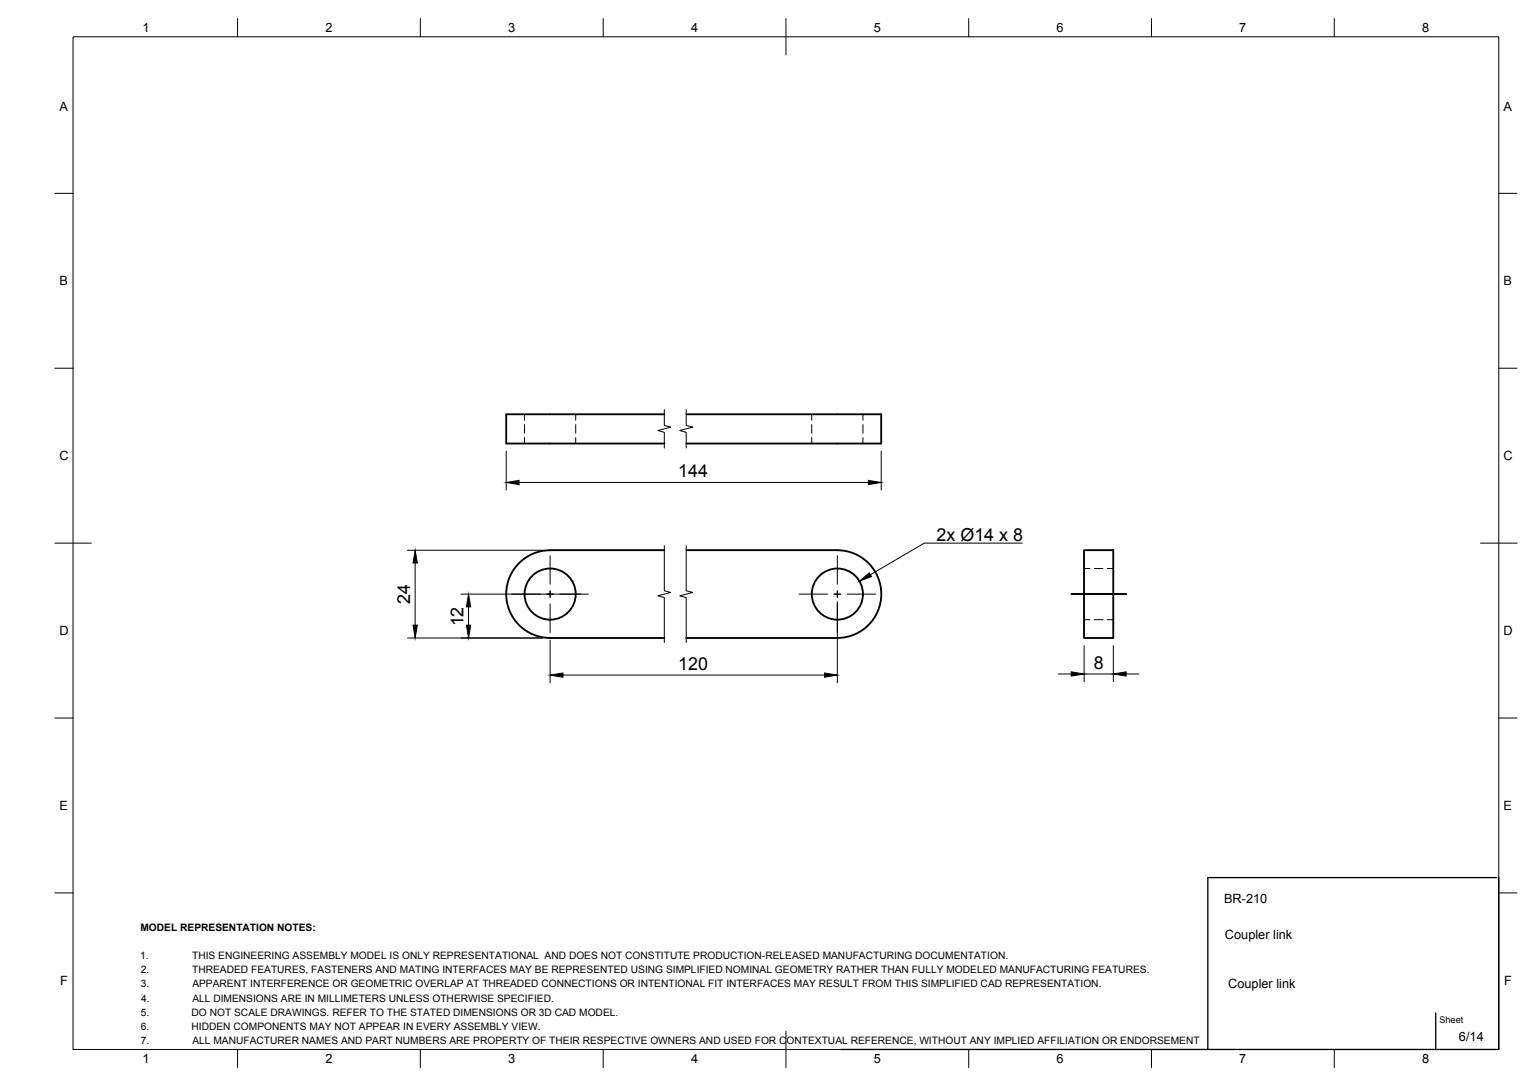
ISO-10303-21;
HEADER;
/* Generated by software containing ST-Developer
 * from STEP Tools, Inc. (www.steptools.com) 
 */

FILE_DESCRIPTION(
/* description */ ('Independent 1:2 reduction pantograph. 120 mm parallelogram sides; fix
ed fulcrum on the extension of a 240 mm link. Drawing point halfway al
ong its link, so its XY displacement is one half of the tracing point.
 Replaceable pivot bushes and retained pins. Calibration and productio
n accuracy unassigned.'),
/* implementation_level */ '2;1');

FILE_NAME(
/* name */ 'Coupler link.step',
/* time_stamp */ '2026-11-07T22:11:57-08:00',
/* author */ (''),
/* organization */ (''),
/* preprocessor_version */ 'ST-DEVELOPER v20.2',
/* originating_system */ 'Autodesk Translation Framework v15.17.0.0',
/* authorisation */ '');

FILE_SCHEMA (('AUTOMOTIVE_DESIGN { 1 0 10303 214 3 1 1 }'));
ENDSEC;

DATA;
#10=MECHANICAL_DESIGN_GEOMETRIC_PRESENTATION_REPRESENTATION('',(#193),#2926);
#167=SHAPE_REPRESENTATION_RELATIONSHIP('SRR','None',#3004,#180);
#180=ADVANCED_BREP_SHAPE_REPRESENTATION('',(#206),#2920);
#193=STYLED_ITEM('',(#3077),#206);
#206=MANIFOLD_SOLID_BREP('Body1',#1548);
#247=FACE_BOUND('',#497,.T.);
#248=FACE_BOUND('',#498,.T.);
#249=FACE_BOUND('',#500,.T.);
#250=FACE_BOUND('',#501,.T.);
#287=PLANE('',#1829);
#288=PLANE('',#1833);
#289=PLANE('',#1837);
#290=PLANE('',#1838);
#363=FACE_OUTER_BOUND('',#490,.T.);
#364=FACE_OUTER_BOUND('',#491,.T.);
#365=FACE_OUTER_BOUND('',#492,.T.);
#366=FACE_OUTER_BOUND('',#493,.T.);
#367=FACE_OUTER_BOUND('',#494,.T.);
#368=FACE_OUTER_BOUND('',#495,.T.);
#369=FACE_OUTER_BOUND('',#496,.T.);
#370=FACE_OUTER_BOUND('',#499,.T.);
#490=EDGE_LOOP('',(#1289,#1290,#1291,#1292));
#491=EDGE_LOOP('',(#1293,#1294,#1295,#1296));
#492=EDGE_LOOP('',(#1297,#1298,#1299,#1300));
#493=EDGE_LOOP('',(#1301,#1302,#1303,#1304));
#494=EDGE_LOOP('',(#1305,#1306,#1307,#1308));
#495=EDGE_LOOP('',(#1309,#1310,#1311,#1312));
#496=EDGE_LOOP('',(#1313,#1314,#1315,#1316));
#497=EDGE_LOOP('',(#1317));
#498=EDGE_LOOP('',(#1318));
#499=EDGE_LOOP('',(#1319,#1320,#1321,#1322));
#500=EDGE_LOOP('',(#1323));
#501=EDGE_LOOP('',(#1324));
#588=LINE('',#2728,#669);
#589=LINE('',#2734,#670);
#590=LINE('',#2739,#671);
#591=LINE('',#2741,#672);
#592=LINE('',#2743,#673);
#593=LINE('',#2744,#674);
#594=LINE('',#2750,#675);
#595=LINE('',#2753,#676);
#596=LINE('',#2755,#677);
#597=LINE('',#2756,#678);
#669=VECTOR('',#2236,7.);
#670=VECTOR('',#2243,7.);
#671=VECTOR('',#2248,10.);
#672=VECTOR('',#2249,10.);
#673=VECTOR('',#2250,10.);
#674=VECTOR('',#2251,10.);
#675=VECTOR('',#2258,10.);
#676=VECTOR('',#2261,10.);
#677=VECTOR('',#2262,10.);
#678=VECTOR('',#2263,10.);
#755=CIRCLE('',#1824,7.);
#756=CIRCLE('',#1825,7.);
#757=CIRCLE('',#1827,7.);
#758=CIRCLE('',#1828,7.);
#759=CIRCLE('',#1831,12.);
#760=CIRCLE('',#1832,12.);
#761=CIRCLE('',#1835,12.);
#762=CIRCLE('',#1836,12.);
#859=VERTEX_POINT('',#2725);
#860=VERTEX_POINT('',#2727);
#861=VERTEX_POINT('',#2731);
#862=VERTEX_POINT('',#2733);
#863=VERTEX_POINT('',#2737);
#864=VERTEX_POINT('',#2738);
#865=VERTEX_POINT('',#2740);
#866=VERTEX_POINT('',#2742);
#867=VERTEX_POINT('',#2746);
#868=VERTEX_POINT('',#2748);
#869=VERTEX_POINT('',#2752);
#870=VERTEX_POINT('',#2754);
#1009=EDGE_CURVE('',#859,#859,#755,.T.);
#1010=EDGE_CURVE('',#859,#860,#588,.T.);
#1011=EDGE_CURVE('',#860,#860,#756,.T.);
#1012=EDGE_CURVE('',#861,#861,#757,.T.);
#1013=EDGE_CURVE('',#861,#862,#589,.T.);
#1014=EDGE_CURVE('',#862,#862,#758,.T.);
#1015=EDGE_CURVE('',#863,#864,#590,.T.);
#1016=EDGE_CURVE('',#864,#865,#591,.T.);
#1017=EDGE_CURVE('',#866,#865,#592,.T.);
#1018=EDGE_CURVE('',#863,#866,#593,.T.);
#1019=EDGE_CURVE('',#867,#863,#759,.T.);
#1020=EDGE_CURVE('',#868,#866,#760,.T.);
#1021=EDGE_CURVE('',#867,#868,#594,.T.);
#1022=EDGE_CURVE('',#869,#867,#595,.T.);
#1023=EDGE_CURVE('',#870,#868,#596,.T.);
#1024=EDGE_CURVE('',#869,#870,#597,.T.);
#1025=EDGE_CURVE('',#864,#869,#761,.T.);
#1026=EDGE_CURVE('',#865,#870,#762,.T.);
#1289=ORIENTED_EDGE('',*,*,#1009,.F.);
#1290=ORIENTED_EDGE('',*,*,#1010,.T.);
#1291=ORIENTED_EDGE('',*,*,#1011,.F.);
#1292=ORIENTED_EDGE('',*,*,#1010,.F.);
#1293=ORIENTED_EDGE('',*,*,#1012,.F.);
#1294=ORIENTED_EDGE('',*,*,#1013,.T.);
#1295=ORIENTED_EDGE('',*,*,#1014,.F.);
#1296=ORIENTED_EDGE('',*,*,#1013,.F.);
#1297=ORIENTED_EDGE('',*,*,#1015,.T.);
#1298=ORIENTED_EDGE('',*,*,#1016,.T.);
#1299=ORIENTED_EDGE('',*,*,#1017,.F.);
#1300=ORIENTED_EDGE('',*,*,#1018,.F.);
#1301=ORIENTED_EDGE('',*,*,#1019,.T.);
#1302=ORIENTED_EDGE('',*,*,#1018,.T.);
#1303=ORIENTED_EDGE('',*,*,#1020,.F.);
#1304=ORIENTED_EDGE('',*,*,#1021,.F.);
#1305=ORIENTED_EDGE('',*,*,#1022,.T.);
#1306=ORIENTED_EDGE('',*,*,#1021,.T.);
#1307=ORIENTED_EDGE('',*,*,#1023,.F.);
#1308=ORIENTED_EDGE('',*,*,#1024,.F.);
#1309=ORIENTED_EDGE('',*,*,#1025,.T.);
#1310=ORIENTED_EDGE('',*,*,#1024,.T.);
#1311=ORIENTED_EDGE('',*,*,#1026,.F.);
#1312=ORIENTED_EDGE('',*,*,#1016,.F.);
#1313=ORIENTED_EDGE('',*,*,#1026,.T.);
#1314=ORIENTED_EDGE('',*,*,#1023,.T.);
#1315=ORIENTED_EDGE('',*,*,#1020,.T.);
#1316=ORIENTED_EDGE('',*,*,#1017,.T.);
#1317=ORIENTED_EDGE('',*,*,#1009,.T.);
#1318=ORIENTED_EDGE('',*,*,#1012,.T.);
#1319=ORIENTED_EDGE('',*,*,#1025,.F.);
#1320=ORIENTED_EDGE('',*,*,#1015,.F.);
#1321=ORIENTED_EDGE('',*,*,#1019,.F.);
#1322=ORIENTED_EDGE('',*,*,#1022,.F.);
#1323=ORIENTED_EDGE('',*,*,#1011,.T.);
#1324=ORIENTED_EDGE('',*,*,#1014,.T.);
#1434=CYLINDRICAL_SURFACE('',#1823,7.);
#1435=CYLINDRICAL_SURFACE('',#1826,7.);
#1436=CYLINDRICAL_SURFACE('',#1830,12.);
#1437=CYLINDRICAL_SURFACE('',#1834,12.);
#1507=ADVANCED_FACE('',(#363),#1434,.F.);
#1508=ADVANCED_FACE('',(#364),#1435,.F.);
#1509=ADVANCED_FACE('',(#365),#287,.T.);
#1510=ADVANCED_FACE('',(#366),#1436,.T.);
#1511=ADVANCED_FACE('',(#367),#288,.T.);
#1512=ADVANCED_FACE('',(#368),#1437,.T.);
#1513=ADVANCED_FACE('',(#369,#247,#248),#289,.T.);
#1514=ADVANCED_FACE('',(#370,#249,#250),#290,.F.);
#1548=CLOSED_SHELL('',(#1507,#1508,#1509,#1510,#1511,#1512,#1513,#1514));
#1822=AXIS2_PLACEMENT_3D('',#2723,#2230,#2231);
#1823=AXIS2_PLACEMENT_3D('',#2724,#2232,#2233);
#1824=AXIS2_PLACEMENT_3D('',#2726,#2234,#2235);
#1825=AXIS2_PLACEMENT_3D('',#2729,#2237,#2238);
#1826=AXIS2_PLACEMENT_3D('',#2730,#2239,#2240);
#1827=AXIS2_PLACEMENT_3D('',#2732,#2241,#2242);
#1828=AXIS2_PLACEMENT_3D('',#2735,#2244,#2245);
#1829=AXIS2_PLACEMENT_3D('',#2736,#2246,#2247);
#1830=AXIS2_PLACEMENT_3D('',#2745,#2252,#2253);
#1831=AXIS2_PLACEMENT_3D('',#2747,#2254,#2255);
#1832=AXIS2_PLACEMENT_3D('',#2749,#2256,#2257);
#1833=AXIS2_PLACEMENT_3D('',#2751,#2259,#2260);
#1834=AXIS2_PLACEMENT_3D('',#2757,#2264,#2265);
#1835=AXIS2_PLACEMENT_3D('',#2758,#2266,#2267);
#1836=AXIS2_PLACEMENT_3D('',#2759,#2268,#2269);
#1837=AXIS2_PLACEMENT_3D('',#2760,#2270,#2271);
#1838=AXIS2_PLACEMENT_3D('',#2761,#2272,#2273);
#2230=DIRECTION('axis',(0.,0.,1.));
#2231=DIRECTION('refdir',(1.,0.,0.));
#2232=DIRECTION('center_axis',(0.,0.,-1.));
#2233=DIRECTION('ref_axis',(1.,0.,0.));
#2234=DIRECTION('center_axis',(0.,0.,-1.));
#2235=DIRECTION('ref_axis',(1.,0.,0.));
#2236=DIRECTION('',(0.,0.,-1.));
#2237=DIRECTION('center_axis',(0.,0.,1.));
#2238=DIRECTION('ref_axis',(1.,0.,0.));
#2239=DIRECTION('center_axis',(0.,0.,-1.));
#2240=DIRECTION('ref_axis',(1.,0.,0.));
#2241=DIRECTION('center_axis',(0.,0.,-1.));
#2242=DIRECTION('ref_axis',(1.,0.,0.));
#2243=DIRECTION('',(0.,0.,-1.));
#2244=DIRECTION('center_axis',(0.,0.,1.));
#2245=DIRECTION('ref_axis',(1.,0.,0.));
#2246=DIRECTION('center_axis',(0.,1.,0.));
#2247=DIRECTION('ref_axis',(-1.,0.,0.));
#2248=DIRECTION('',(-1.,0.,0.));
#2249=DIRECTION('',(0.,0.,1.));
#2250=DIRECTION('',(-1.,0.,0.));
#2251=DIRECTION('',(0.,0.,1.));
#2252=DIRECTION('center_axis',(0.,0.,1.));
#2253=DIRECTION('ref_axis',(0.,-1.,0.));
#2254=DIRECTION('center_axis',(0.,0.,1.));
#2255=DIRECTION('ref_axis',(0.,-1.,0.));
#2256=DIRECTION('center_axis',(0.,0.,1.));
#2257=DIRECTION('ref_axis',(0.,-1.,0.));
#2258=DIRECTION('',(0.,0.,1.));
#2259=DIRECTION('center_axis',(0.,-1.,0.));
#2260=DIRECTION('ref_axis',(1.,0.,0.));
#2261=DIRECTION('',(1.,0.,0.));
#2262=DIRECTION('',(1.,0.,0.));
#2263=DIRECTION('',(0.,0.,1.));
#2264=DIRECTION('center_axis',(0.,0.,1.));
#2265=DIRECTION('ref_axis',(0.,1.,0.));
#2266=DIRECTION('center_axis',(0.,0.,1.));
#2267=DIRECTION('ref_axis',(0.,1.,0.));
#2268=DIRECTION('center_axis',(0.,0.,1.));
#2269=DIRECTION('ref_axis',(0.,1.,0.));
#2270=DIRECTION('center_axis',(0.,0.,1.));
#2271=DIRECTION('ref_axis',(1.,0.,0.));
#2272=DIRECTION('center_axis',(0.,0.,1.));
#2273=DIRECTION('ref_axis',(1.,0.,0.));
#2723=CARTESIAN_POINT('',(0.,0.,0.));
#2724=CARTESIAN_POINT('Origin',(0.,0.,4.));
#2725=CARTESIAN_POINT('',(-7.,8.57252759403147E-16,8.));
#2726=CARTESIAN_POINT('Origin',(0.,0.,8.));
#2727=CARTESIAN_POINT('',(-7.,8.57252759403147E-16,0.));
#2728=CARTESIAN_POINT('',(-7.,8.57252759403147E-16,4.));
#2729=CARTESIAN_POINT('Origin',(0.,0.,0.));
#2730=CARTESIAN_POINT('Origin',(120.,0.,4.));
#2731=CARTESIAN_POINT('',(113.,8.57252759403147E-16,8.));
#2732=CARTESIAN_POINT('Origin',(120.,0.,8.));
#2733=CARTESIAN_POINT('',(113.,8.57252759403147E-16,0.));
#2734=CARTESIAN_POINT('',(113.,8.57252759403147E-16,4.));
#2735=CARTESIAN_POINT('Origin',(120.,0.,0.));
#2736=CARTESIAN_POINT('Origin',(120.,12.,0.));
#2737=CARTESIAN_POINT('',(120.,12.,0.));
#2738=CARTESIAN_POINT('',(0.,12.,0.));
#2739=CARTESIAN_POINT('',(120.,12.,0.));
#2740=CARTESIAN_POINT('',(0.,12.,8.));
#2741=CARTESIAN_POINT('',(0.,12.,0.));
#2742=CARTESIAN_POINT('',(120.,12.,8.));
#2743=CARTESIAN_POINT('',(120.,12.,8.));
#2744=CARTESIAN_POINT('',(120.,12.,0.));
#2745=CARTESIAN_POINT('Origin',(120.,-1.11022302462516E-15,0.));
#2746=CARTESIAN_POINT('',(120.,-12.,0.));
#2747=CARTESIAN_POINT('Origin',(120.,-1.11022302462516E-15,0.));
#2748=CARTESIAN_POINT('',(120.,-12.,8.));
#2749=CARTESIAN_POINT('Origin',(120.,-1.11022302462516E-15,8.));
#2750=CARTESIAN_POINT('',(120.,-12.,0.));
#2751=CARTESIAN_POINT('Origin',(0.,-12.,0.));
#2752=CARTESIAN_POINT('',(-1.46957615897682E-15,-12.,0.));
#2753=CARTESIAN_POINT('',(0.,-12.,0.));
#2754=CARTESIAN_POINT('',(-1.46957615897682E-15,-12.,8.));
#2755=CARTESIAN_POINT('',(0.,-12.,8.));
#2756=CARTESIAN_POINT('',(-1.46957615897682E-15,-12.,0.));
#2757=CARTESIAN_POINT('Origin',(0.,0.,0.));
#2758=CARTESIAN_POINT('Origin',(0.,0.,0.));
#2759=CARTESIAN_POINT('Origin',(0.,0.,8.));
#2760=CARTESIAN_POINT('Origin',(60.,0.,8.));
#2761=CARTESIAN_POINT('Origin',(60.,0.,0.));
#2905=UNCERTAINTY_MEASURE_WITH_UNIT(LENGTH_MEASURE(0.01),#2927,
'DISTANCE_ACCURACY_VALUE',
'Maximum model space distance between geometric entities at asserted c
onnectivities');
#2911=UNCERTAINTY_MEASURE_WITH_UNIT(LENGTH_MEASURE(0.01),#2927,
'DISTANCE_ACCURACY_VALUE',
'Maximum model space distance between geometric entities at asserted c
onnectivities');
#2920=(
GEOMETRIC_REPRESENTATION_CONTEXT(3)
GLOBAL_UNCERTAINTY_ASSIGNED_CONTEXT((#2905))
GLOBAL_UNIT_ASSIGNED_CONTEXT((#2927,#2929,#2930))
REPRESENTATION_CONTEXT('','3D')
);
#2926=(
GEOMETRIC_REPRESENTATION_CONTEXT(3)
GLOBAL_UNCERTAINTY_ASSIGNED_CONTEXT((#2911))
GLOBAL_UNIT_ASSIGNED_CONTEXT((#2927,#2929,#2930))
REPRESENTATION_CONTEXT('','3D')
);
#2927=(
LENGTH_UNIT()
NAMED_UNIT(*)
SI_UNIT(.MILLI.,.METRE.)
);
#2929=(
NAMED_UNIT(*)
PLANE_ANGLE_UNIT()
SI_UNIT($,.RADIAN.)
);
#2930=(
NAMED_UNIT(*)
SI_UNIT($,.STERADIAN.)
SOLID_ANGLE_UNIT()
);
#2939=SHAPE_DEFINITION_REPRESENTATION(#2953,#3004);
#2953=PRODUCT_DEFINITION_SHAPE('',$,#3019);
#3004=SHAPE_REPRESENTATION('',(#1822),#2920);
#3010=PRODUCT_DEFINITION_CONTEXT('part definition',#3054,'design');
#3019=PRODUCT_DEFINITION('Coupler link','Coupler link',#3033,#3010);
#3033=PRODUCT_DEFINITION_FORMATION('',$,#3064);
#3054=APPLICATION_CONTEXT(
'Core Data for Automotive Mechanical Design Process');
#3055=PRODUCT_CONTEXT('part definition',#3054,'mechanical');
#3064=PRODUCT('Coupler link','Coupler link',$,(#3055));
#3077=PRESENTATION_STYLE_ASSIGNMENT((#3089));
#3089=SURFACE_STYLE_USAGE(.BOTH.,#3101);
#3101=SURFACE_SIDE_STYLE('',(#3113));
#3113=SURFACE_STYLE_FILL_AREA(#3125);
#3125=FILL_AREA_STYLE('Coupler link finish',(#3137));
#3137=FILL_AREA_STYLE_COLOUR('Coupler link finish',#3149);
#3149=COLOUR_RGB('Coupler link finish',0.317647058823529,0.686274509803922,
0.890196078431372);
ENDSEC;
END-ISO-10303-21;
